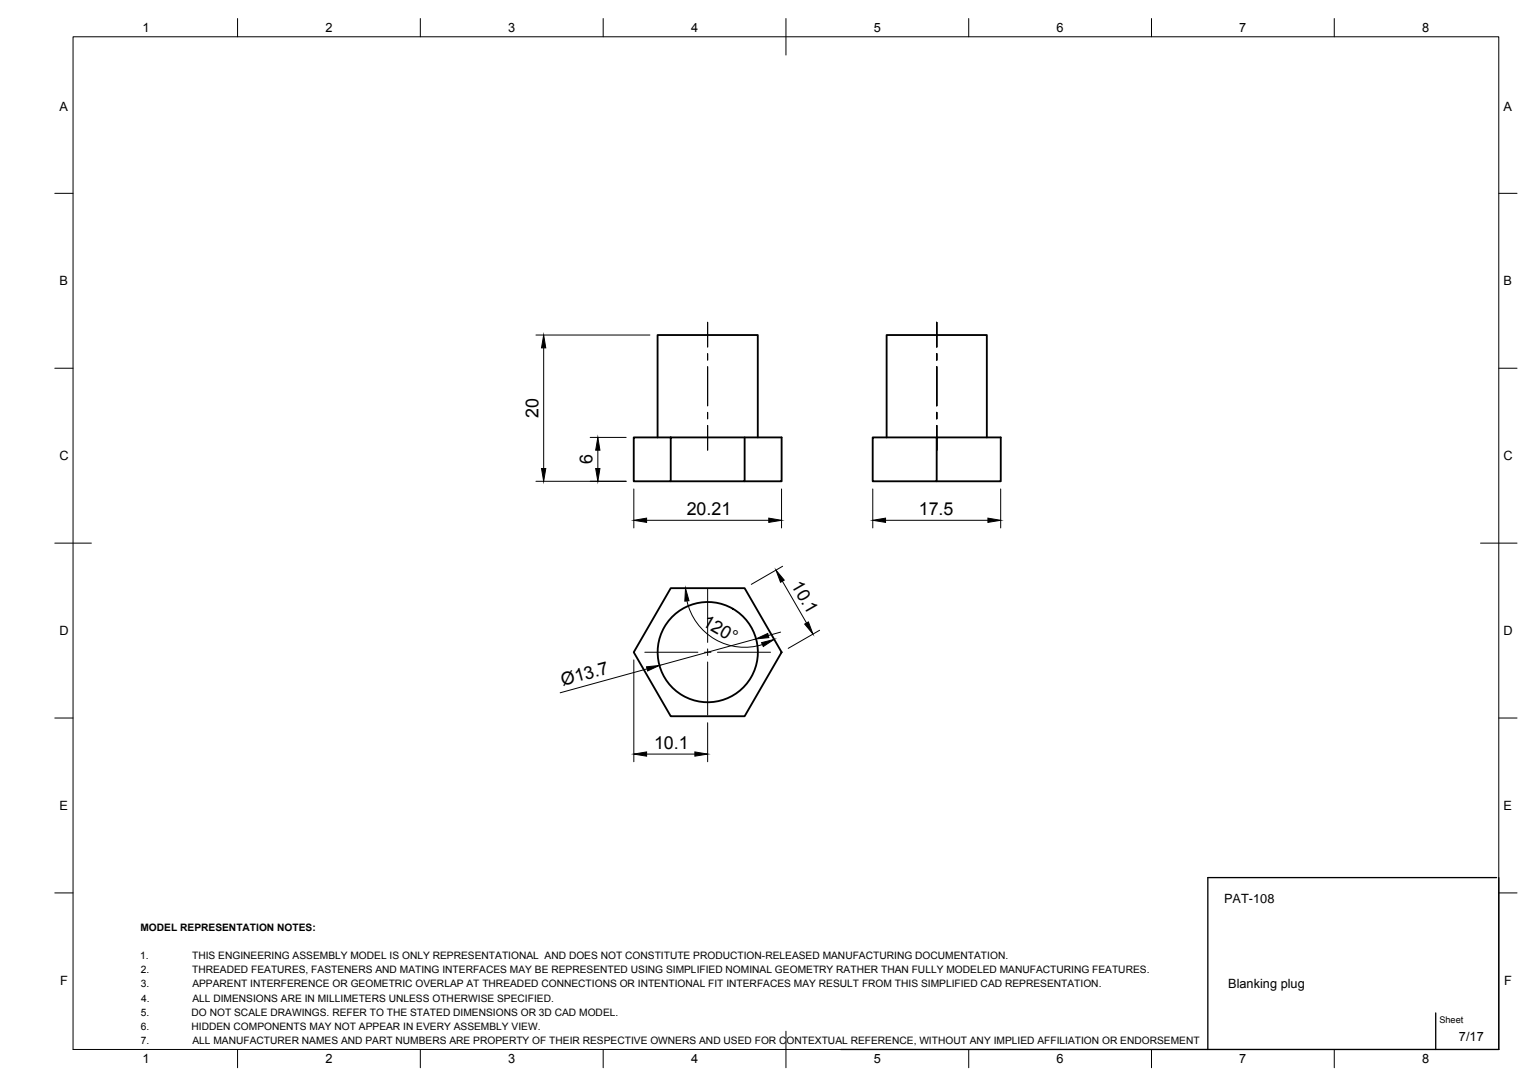
ISO-10303-21;
HEADER;
/* Generated by software containing ST-Developer
 * from STEP Tools, Inc. (www.steptools.com) 
 */

FILE_DESCRIPTION(
/* description */ ('Sub-base valve envelopes and connections'),
/* implementation_level */ '2;1');

FILE_NAME(
/* name */ 'Blanking plug.step',
/* time_stamp */ '2026-10-29T15:55:44-07:00',
/* author */ (''),
/* organization */ (''),
/* preprocessor_version */ 'ST-DEVELOPER v20.2',
/* originating_system */ 'Autodesk Translation Framework v15.17.0.0',
/* authorisation */ '');

FILE_SCHEMA (('AUTOMOTIVE_DESIGN { 1 0 10303 214 3 1 1 }'));
ENDSEC;

DATA;
#10=MECHANICAL_DESIGN_GEOMETRIC_PRESENTATION_REPRESENTATION('',(#123),#6113);
#99=SHAPE_REPRESENTATION_RELATIONSHIP('SRR','None',#6172,#111);
#111=ADVANCED_BREP_SHAPE_REPRESENTATION('',(#135),#6103);
#123=STYLED_ITEM('',(#6329),#135);
#135=MANIFOLD_SOLID_BREP('Body1',#3362);
#210=FACE_BOUND('',#746,.T.);
#317=PLANE('',#3698);
#318=PLANE('',#3700);
#319=PLANE('',#3701);
#320=PLANE('',#3702);
#321=PLANE('',#3703);
#322=PLANE('',#3704);
#323=PLANE('',#3705);
#324=PLANE('',#3706);
#325=PLANE('',#3709);
#478=FACE_OUTER_BOUND('',#745,.T.);
#479=FACE_OUTER_BOUND('',#747,.T.);
#480=FACE_OUTER_BOUND('',#748,.T.);
#481=FACE_OUTER_BOUND('',#749,.T.);
#482=FACE_OUTER_BOUND('',#750,.T.);
#483=FACE_OUTER_BOUND('',#751,.T.);
#484=FACE_OUTER_BOUND('',#752,.T.);
#485=FACE_OUTER_BOUND('',#753,.T.);
#486=FACE_OUTER_BOUND('',#754,.T.);
#487=FACE_OUTER_BOUND('',#755,.T.);
#745=EDGE_LOOP('',(#2639,#2640,#2641,#2642,#2643,#2644));
#746=EDGE_LOOP('',(#2645));
#747=EDGE_LOOP('',(#2646,#2647,#2648,#2649));
#748=EDGE_LOOP('',(#2650,#2651,#2652,#2653));
#749=EDGE_LOOP('',(#2654,#2655,#2656,#2657));
#750=EDGE_LOOP('',(#2658,#2659,#2660,#2661));
#751=EDGE_LOOP('',(#2662,#2663,#2664,#2665));
#752=EDGE_LOOP('',(#2666,#2667,#2668,#2669));
#753=EDGE_LOOP('',(#2670,#2671,#2672,#2673,#2674,#2675));
#754=EDGE_LOOP('',(#2676,#2677,#2678,#2679));
#755=EDGE_LOOP('',(#2680));
#989=LINE('',#5588,#1223);
#990=LINE('',#5590,#1224);
#991=LINE('',#5592,#1225);
#992=LINE('',#5594,#1226);
#993=LINE('',#5596,#1227);
#994=LINE('',#5597,#1228);
#995=LINE('',#5602,#1229);
#996=LINE('',#5604,#1230);
#997=LINE('',#5605,#1231);
#998=LINE('',#5608,#1232);
#999=LINE('',#5609,#1233);
#1000=LINE('',#5612,#1234);
#1001=LINE('',#5613,#1235);
#1002=LINE('',#5616,#1236);
#1003=LINE('',#5617,#1237);
#1004=LINE('',#5620,#1238);
#1005=LINE('',#5621,#1239);
#1006=LINE('',#5623,#1240);
#1007=LINE('',#5627,#1241);
#1223=VECTOR('',#4383,1.);
#1224=VECTOR('',#4384,1.);
#1225=VECTOR('',#4385,1.);
#1226=VECTOR('',#4386,1.);
#1227=VECTOR('',#4387,1.);
#1228=VECTOR('',#4388,1.);
#1229=VECTOR('',#4393,1.);
#1230=VECTOR('',#4394,1.);
#1231=VECTOR('',#4395,1.);
#1232=VECTOR('',#4398,1.);
#1233=VECTOR('',#4399,1.);
#1234=VECTOR('',#4402,1.);
#1235=VECTOR('',#4403,1.);
#1236=VECTOR('',#4406,1.);
#1237=VECTOR('',#4407,1.);
#1238=VECTOR('',#4410,1.);
#1239=VECTOR('',#4411,1.);
#1240=VECTOR('',#4414,1.);
#1241=VECTOR('',#4419,0.685);
#1465=CIRCLE('',#3699,0.685);
#1466=CIRCLE('',#3708,0.685);
#1671=VERTEX_POINT('',#5586);
#1672=VERTEX_POINT('',#5587);
#1673=VERTEX_POINT('',#5589);
#1674=VERTEX_POINT('',#5591);
#1675=VERTEX_POINT('',#5593);
#1676=VERTEX_POINT('',#5595);
#1677=VERTEX_POINT('',#5598);
#1678=VERTEX_POINT('',#5601);
#1679=VERTEX_POINT('',#5603);
#1680=VERTEX_POINT('',#5607);
#1681=VERTEX_POINT('',#5611);
#1682=VERTEX_POINT('',#5615);
#1683=VERTEX_POINT('',#5619);
#1684=VERTEX_POINT('',#5626);
#2017=EDGE_CURVE('',#1671,#1672,#989,.T.);
#2018=EDGE_CURVE('',#1673,#1671,#990,.T.);
#2019=EDGE_CURVE('',#1674,#1673,#991,.T.);
#2020=EDGE_CURVE('',#1675,#1674,#992,.T.);
#2021=EDGE_CURVE('',#1676,#1675,#993,.T.);
#2022=EDGE_CURVE('',#1672,#1676,#994,.T.);
#2023=EDGE_CURVE('',#1677,#1677,#1465,.T.);
#2024=EDGE_CURVE('',#1671,#1678,#995,.T.);
#2025=EDGE_CURVE('',#1679,#1678,#996,.T.);
#2026=EDGE_CURVE('',#1673,#1679,#997,.T.);
#2027=EDGE_CURVE('',#1680,#1679,#998,.T.);
#2028=EDGE_CURVE('',#1674,#1680,#999,.T.);
#2029=EDGE_CURVE('',#1681,#1680,#1000,.T.);
#2030=EDGE_CURVE('',#1675,#1681,#1001,.T.);
#2031=EDGE_CURVE('',#1682,#1681,#1002,.T.);
#2032=EDGE_CURVE('',#1676,#1682,#1003,.T.);
#2033=EDGE_CURVE('',#1683,#1682,#1004,.T.);
#2034=EDGE_CURVE('',#1672,#1683,#1005,.T.);
#2035=EDGE_CURVE('',#1678,#1683,#1006,.T.);
#2036=EDGE_CURVE('',#1677,#1684,#1007,.T.);
#2037=EDGE_CURVE('',#1684,#1684,#1466,.T.);
#2639=ORIENTED_EDGE('',*,*,#2017,.F.);
#2640=ORIENTED_EDGE('',*,*,#2018,.F.);
#2641=ORIENTED_EDGE('',*,*,#2019,.F.);
#2642=ORIENTED_EDGE('',*,*,#2020,.F.);
#2643=ORIENTED_EDGE('',*,*,#2021,.F.);
#2644=ORIENTED_EDGE('',*,*,#2022,.F.);
#2645=ORIENTED_EDGE('',*,*,#2023,.T.);
#2646=ORIENTED_EDGE('',*,*,#2018,.T.);
#2647=ORIENTED_EDGE('',*,*,#2024,.T.);
#2648=ORIENTED_EDGE('',*,*,#2025,.F.);
#2649=ORIENTED_EDGE('',*,*,#2026,.F.);
#2650=ORIENTED_EDGE('',*,*,#2019,.T.);
#2651=ORIENTED_EDGE('',*,*,#2026,.T.);
#2652=ORIENTED_EDGE('',*,*,#2027,.F.);
#2653=ORIENTED_EDGE('',*,*,#2028,.F.);
#2654=ORIENTED_EDGE('',*,*,#2020,.T.);
#2655=ORIENTED_EDGE('',*,*,#2028,.T.);
#2656=ORIENTED_EDGE('',*,*,#2029,.F.);
#2657=ORIENTED_EDGE('',*,*,#2030,.F.);
#2658=ORIENTED_EDGE('',*,*,#2021,.T.);
#2659=ORIENTED_EDGE('',*,*,#2030,.T.);
#2660=ORIENTED_EDGE('',*,*,#2031,.F.);
#2661=ORIENTED_EDGE('',*,*,#2032,.F.);
#2662=ORIENTED_EDGE('',*,*,#2022,.T.);
#2663=ORIENTED_EDGE('',*,*,#2032,.T.);
#2664=ORIENTED_EDGE('',*,*,#2033,.F.);
#2665=ORIENTED_EDGE('',*,*,#2034,.F.);
#2666=ORIENTED_EDGE('',*,*,#2017,.T.);
#2667=ORIENTED_EDGE('',*,*,#2034,.T.);
#2668=ORIENTED_EDGE('',*,*,#2035,.F.);
#2669=ORIENTED_EDGE('',*,*,#2024,.F.);
#2670=ORIENTED_EDGE('',*,*,#2035,.T.);
#2671=ORIENTED_EDGE('',*,*,#2033,.T.);
#2672=ORIENTED_EDGE('',*,*,#2031,.T.);
#2673=ORIENTED_EDGE('',*,*,#2029,.T.);
#2674=ORIENTED_EDGE('',*,*,#2027,.T.);
#2675=ORIENTED_EDGE('',*,*,#2025,.T.);
#2676=ORIENTED_EDGE('',*,*,#2023,.F.);
#2677=ORIENTED_EDGE('',*,*,#2036,.T.);
#2678=ORIENTED_EDGE('',*,*,#2037,.T.);
#2679=ORIENTED_EDGE('',*,*,#2036,.F.);
#2680=ORIENTED_EDGE('',*,*,#2037,.F.);
#3125=CYLINDRICAL_SURFACE('',#3707,0.685);
#3251=ADVANCED_FACE('',(#478,#210),#317,.F.);
#3252=ADVANCED_FACE('',(#479),#318,.T.);
#3253=ADVANCED_FACE('',(#480),#319,.T.);
#3254=ADVANCED_FACE('',(#481),#320,.T.);
#3255=ADVANCED_FACE('',(#482),#321,.T.);
#3256=ADVANCED_FACE('',(#483),#322,.T.);
#3257=ADVANCED_FACE('',(#484),#323,.T.);
#3258=ADVANCED_FACE('',(#485),#324,.T.);
#3259=ADVANCED_FACE('',(#486),#3125,.T.);
#3260=ADVANCED_FACE('',(#487),#325,.F.);
#3362=CLOSED_SHELL('',(#3251,#3252,#3253,#3254,#3255,#3256,#3257,#3258,
#3259,#3260));
#3697=AXIS2_PLACEMENT_3D('',#5584,#4379,#4380);
#3698=AXIS2_PLACEMENT_3D('',#5585,#4381,#4382);
#3699=AXIS2_PLACEMENT_3D('',#5599,#4389,#4390);
#3700=AXIS2_PLACEMENT_3D('',#5600,#4391,#4392);
#3701=AXIS2_PLACEMENT_3D('',#5606,#4396,#4397);
#3702=AXIS2_PLACEMENT_3D('',#5610,#4400,#4401);
#3703=AXIS2_PLACEMENT_3D('',#5614,#4404,#4405);
#3704=AXIS2_PLACEMENT_3D('',#5618,#4408,#4409);
#3705=AXIS2_PLACEMENT_3D('',#5622,#4412,#4413);
#3706=AXIS2_PLACEMENT_3D('',#5624,#4415,#4416);
#3707=AXIS2_PLACEMENT_3D('',#5625,#4417,#4418);
#3708=AXIS2_PLACEMENT_3D('',#5628,#4420,#4421);
#3709=AXIS2_PLACEMENT_3D('',#5629,#4422,#4423);
#4379=DIRECTION('axis',(0.,0.,1.));
#4380=DIRECTION('refdir',(1.,0.,0.));
#4381=DIRECTION('center_axis',(1.,0.,0.));
#4382=DIRECTION('ref_axis',(0.,0.,-1.));
#4383=DIRECTION('',(0.,0.5,0.866025403784439));
#4384=DIRECTION('',(0.,1.,-4.39534328316243E-16));
#4385=DIRECTION('',(0.,0.5,-0.866025403784439));
#4386=DIRECTION('',(0.,-0.5,-0.866025403784439));
#4387=DIRECTION('',(0.,-1.,0.));
#4388=DIRECTION('',(0.,-0.5,0.866025403784439));
#4389=DIRECTION('center_axis',(1.,0.,0.));
#4390=DIRECTION('ref_axis',(0.,0.,-1.));
#4391=DIRECTION('center_axis',(0.,-4.39534328316243E-16,-1.));
#4392=DIRECTION('ref_axis',(0.,1.,-4.39534328316243E-16));
#4393=DIRECTION('',(1.,0.,0.));
#4394=DIRECTION('',(0.,1.,-4.39534328316243E-16));
#4395=DIRECTION('',(1.,0.,0.));
#4396=DIRECTION('center_axis',(0.,-0.866025403784439,-0.5));
#4397=DIRECTION('ref_axis',(0.,0.5,-0.866025403784439));
#4398=DIRECTION('',(0.,0.5,-0.866025403784439));
#4399=DIRECTION('',(1.,0.,0.));
#4400=DIRECTION('center_axis',(0.,-0.866025403784439,0.5));
#4401=DIRECTION('ref_axis',(0.,-0.5,-0.866025403784439));
#4402=DIRECTION('',(0.,-0.5,-0.866025403784439));
#4403=DIRECTION('',(1.,0.,0.));
#4404=DIRECTION('center_axis',(0.,0.,1.));
#4405=DIRECTION('ref_axis',(0.,-1.,0.));
#4406=DIRECTION('',(0.,-1.,0.));
#4407=DIRECTION('',(1.,0.,0.));
#4408=DIRECTION('center_axis',(0.,0.866025403784439,0.5));
#4409=DIRECTION('ref_axis',(0.,-0.5,0.866025403784439));
#4410=DIRECTION('',(0.,-0.5,0.866025403784439));
#4411=DIRECTION('',(1.,0.,0.));
#4412=DIRECTION('center_axis',(0.,0.866025403784439,-0.5));
#4413=DIRECTION('ref_axis',(0.,0.5,0.866025403784439));
#4414=DIRECTION('',(0.,0.5,0.866025403784439));
#4415=DIRECTION('center_axis',(1.,0.,0.));
#4416=DIRECTION('ref_axis',(0.,0.,-1.));
#4417=DIRECTION('center_axis',(1.,0.,0.));
#4418=DIRECTION('ref_axis',(0.,0.,-1.));
#4419=DIRECTION('',(-1.,0.,0.));
#4420=DIRECTION('center_axis',(1.,0.,0.));
#4421=DIRECTION('ref_axis',(0.,0.,-1.));
#4422=DIRECTION('center_axis',(1.,0.,0.));
#4423=DIRECTION('ref_axis',(0.,0.,-1.));
#5584=CARTESIAN_POINT('',(0.,0.,0.));
#5585=CARTESIAN_POINT('Origin',(5.5,0.,3.5));
#5586=CARTESIAN_POINT('',(5.5,0.505181485540923,2.625));
#5587=CARTESIAN_POINT('',(5.5,1.01036297108185,3.5));
#5588=CARTESIAN_POINT('',(5.5,0.505181485540923,2.625));
#5589=CARTESIAN_POINT('',(5.5,-0.505181485540923,2.625));
#5590=CARTESIAN_POINT('',(5.5,-0.505181485540923,2.625));
#5591=CARTESIAN_POINT('',(5.5,-1.01036297108185,3.5));
#5592=CARTESIAN_POINT('',(5.5,-1.01036297108185,3.5));
#5593=CARTESIAN_POINT('',(5.5,-0.505181485540922,4.375));
#5594=CARTESIAN_POINT('',(5.5,-0.505181485540922,4.375));
#5595=CARTESIAN_POINT('',(5.5,0.505181485540923,4.375));
#5596=CARTESIAN_POINT('',(5.5,0.505181485540923,4.375));
#5597=CARTESIAN_POINT('',(5.5,1.01036297108185,3.5));
#5598=CARTESIAN_POINT('',(5.5,-8.38883057415937E-17,4.185));
#5599=CARTESIAN_POINT('Origin',(5.5,0.,3.5));
#5600=CARTESIAN_POINT('Origin',(5.5,-0.505181485540923,2.625));
#5601=CARTESIAN_POINT('',(6.1,0.505181485540923,2.625));
#5602=CARTESIAN_POINT('',(5.5,0.505181485540923,2.625));
#5603=CARTESIAN_POINT('',(6.1,-0.505181485540923,2.625));
#5604=CARTESIAN_POINT('',(6.1,-0.505181485540923,2.625));
#5605=CARTESIAN_POINT('',(5.5,-0.505181485540923,2.625));
#5606=CARTESIAN_POINT('Origin',(5.5,-1.01036297108185,3.5));
#5607=CARTESIAN_POINT('',(6.1,-1.01036297108185,3.5));
#5608=CARTESIAN_POINT('',(6.1,-1.01036297108185,3.5));
#5609=CARTESIAN_POINT('',(5.5,-1.01036297108185,3.5));
#5610=CARTESIAN_POINT('Origin',(5.5,-0.505181485540922,4.375));
#5611=CARTESIAN_POINT('',(6.1,-0.505181485540922,4.375));
#5612=CARTESIAN_POINT('',(6.1,-0.505181485540922,4.375));
#5613=CARTESIAN_POINT('',(5.5,-0.505181485540922,4.375));
#5614=CARTESIAN_POINT('Origin',(5.5,0.505181485540923,4.375));
#5615=CARTESIAN_POINT('',(6.1,0.505181485540923,4.375));
#5616=CARTESIAN_POINT('',(6.1,0.505181485540923,4.375));
#5617=CARTESIAN_POINT('',(5.5,0.505181485540923,4.375));
#5618=CARTESIAN_POINT('Origin',(5.5,1.01036297108185,3.5));
#5619=CARTESIAN_POINT('',(6.1,1.01036297108185,3.5));
#5620=CARTESIAN_POINT('',(6.1,1.01036297108185,3.5));
#5621=CARTESIAN_POINT('',(5.5,1.01036297108185,3.5));
#5622=CARTESIAN_POINT('Origin',(5.5,0.505181485540923,2.625));
#5623=CARTESIAN_POINT('',(6.1,0.505181485540923,2.625));
#5624=CARTESIAN_POINT('Origin',(6.1,0.,3.5));
#5625=CARTESIAN_POINT('Origin',(4.1,0.,3.5));
#5626=CARTESIAN_POINT('',(4.1,-8.38883057415937E-17,4.185));
#5627=CARTESIAN_POINT('',(4.1,-8.38883057415937E-17,4.185));
#5628=CARTESIAN_POINT('Origin',(4.1,0.,3.5));
#5629=CARTESIAN_POINT('Origin',(4.1,0.,3.5));
#6087=UNCERTAINTY_MEASURE_WITH_UNIT(LENGTH_MEASURE(0.001),#6114,
'DISTANCE_ACCURACY_VALUE',
'Maximum model space distance between geometric entities at asserted c
onnectivities');
#6097=UNCERTAINTY_MEASURE_WITH_UNIT(LENGTH_MEASURE(0.001),#6114,
'DISTANCE_ACCURACY_VALUE',
'Maximum model space distance between geometric entities at asserted c
onnectivities');
#6103=(
GEOMETRIC_REPRESENTATION_CONTEXT(3)
GLOBAL_UNCERTAINTY_ASSIGNED_CONTEXT((#6087))
GLOBAL_UNIT_ASSIGNED_CONTEXT((#6114,#6116,#6117))
REPRESENTATION_CONTEXT('','3D')
);
#6113=(
GEOMETRIC_REPRESENTATION_CONTEXT(3)
GLOBAL_UNCERTAINTY_ASSIGNED_CONTEXT((#6097))
GLOBAL_UNIT_ASSIGNED_CONTEXT((#6114,#6116,#6117))
REPRESENTATION_CONTEXT('','3D')
);
#6114=(
LENGTH_UNIT()
NAMED_UNIT(*)
SI_UNIT(.CENTI.,.METRE.)
);
#6116=(
NAMED_UNIT(*)
PLANE_ANGLE_UNIT()
SI_UNIT($,.RADIAN.)
);
#6117=(
NAMED_UNIT(*)
SI_UNIT($,.STERADIAN.)
SOLID_ANGLE_UNIT()
);
#6123=SHAPE_DEFINITION_REPRESENTATION(#6138,#6172);
#6138=PRODUCT_DEFINITION_SHAPE('',$,#6188);
#6172=SHAPE_REPRESENTATION('',(#3697),#6103);
#6182=PRODUCT_DEFINITION_CONTEXT('part definition',#6229,'design');
#6188=PRODUCT_DEFINITION('Blanking plug','Blanking plug',#6203,
#6182);
#6203=PRODUCT_DEFINITION_FORMATION('',$,#6236);
#6229=APPLICATION_CONTEXT(
'Core Data for Automotive Mechanical Design Process');
#6230=PRODUCT_CONTEXT('part definition',#6229,'mechanical');
#6236=PRODUCT('Blanking plug','Blanking plug',
'Blanking plug',(#6230));
#6323=COLOUR_RGB('Off White',0.89,0.88,0.83);
#6324=FILL_AREA_STYLE_COLOUR('',#6323);
#6325=FILL_AREA_STYLE('',(#6324));
#6326=SURFACE_STYLE_FILL_AREA(#6325);
#6327=SURFACE_SIDE_STYLE('',(#6326));
#6328=SURFACE_STYLE_USAGE(.BOTH.,#6327);
#6329=PRESENTATION_STYLE_ASSIGNMENT((#6328));
ENDSEC;
END-ISO-10303-21;
